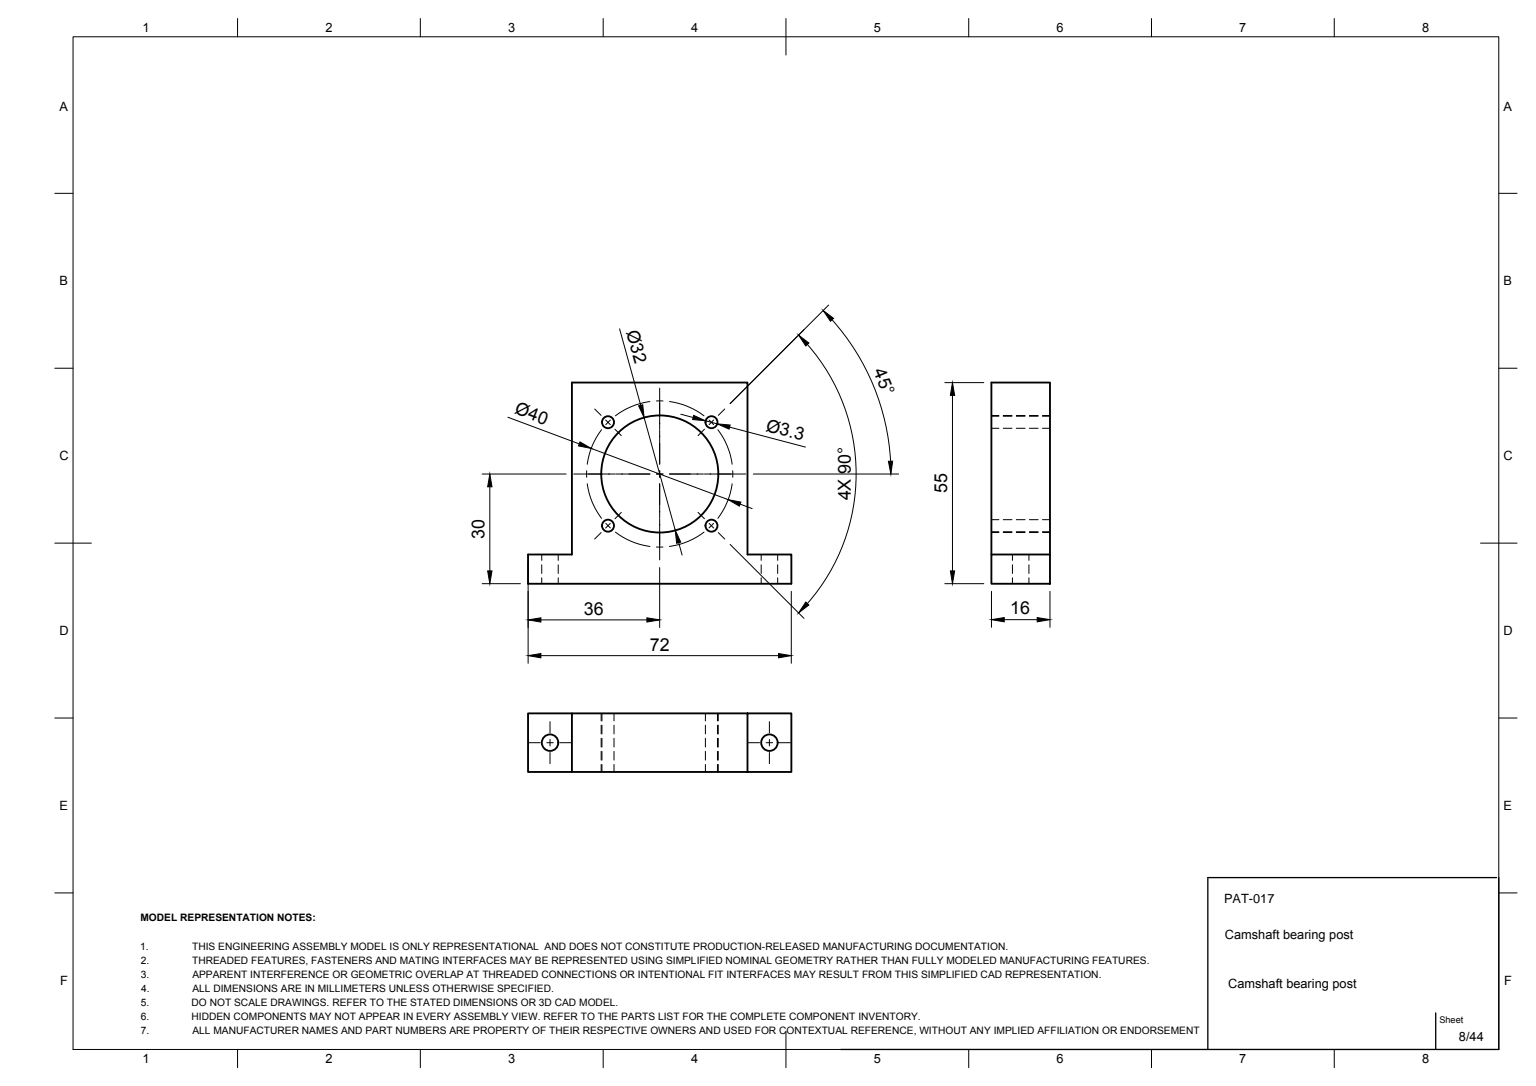
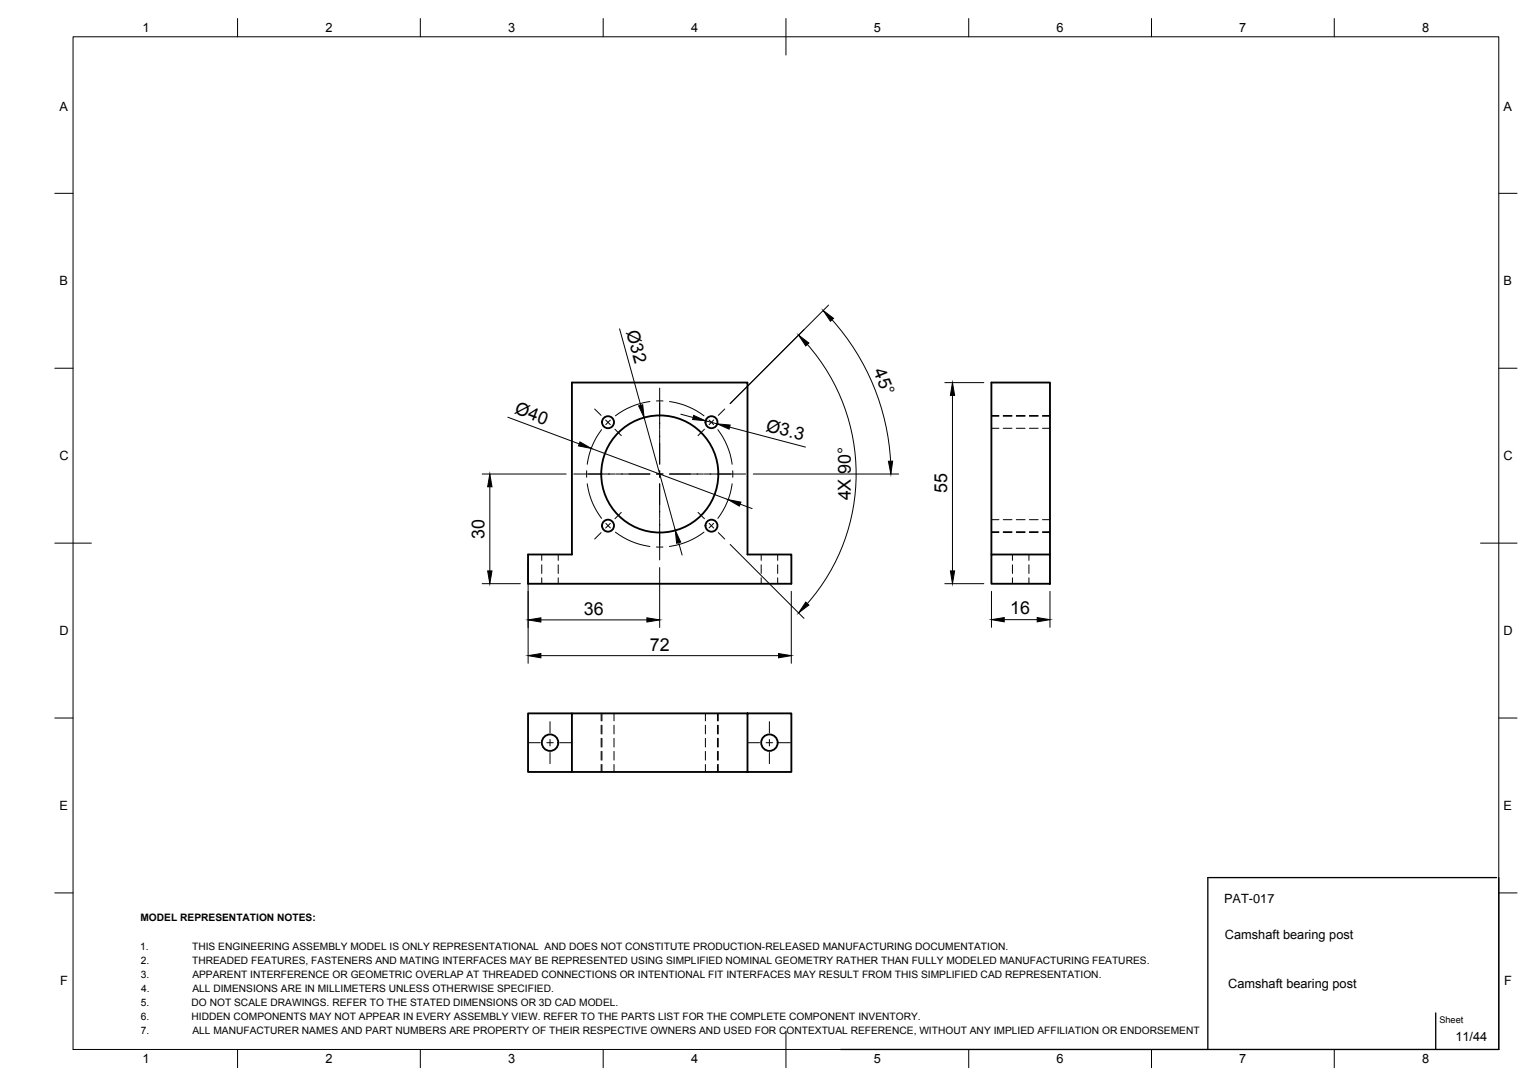
ISO-10303-21;
HEADER;
/* Generated by software containing ST-Developer
 * from STEP Tools, Inc. (www.steptools.com) 
 */

FILE_DESCRIPTION(
/* description */ ('Cam-and-follower valve demonstrator'),
/* implementation_level */ '2;1');

FILE_NAME(
/* name */ 'Camshaft bearing post.step',
/* time_stamp */ '2026-10-28T03:25:17-07:00',
/* author */ (''),
/* organization */ (''),
/* preprocessor_version */ 'ST-DEVELOPER v20.2',
/* originating_system */ 'Autodesk Translation Framework v15.17.0.0',
/* authorisation */ '');

FILE_SCHEMA (('AUTOMOTIVE_DESIGN { 1 0 10303 214 3 1 1 }'));
ENDSEC;

DATA;
#10=MECHANICAL_DESIGN_GEOMETRIC_PRESENTATION_REPRESENTATION('',(#415),#12896);
#343=SHAPE_REPRESENTATION_RELATIONSHIP('SRR','None',#13059,#379);
#379=ADVANCED_BREP_SHAPE_REPRESENTATION('',(#458),#12859);
#415=STYLED_ITEM('',(#13330),#458);
#458=MANIFOLD_SOLID_BREP('Body1',#6182);
#508=FACE_BOUND('',#1513,.T.);
#509=FACE_BOUND('',#1515,.T.);
#510=FACE_BOUND('',#1519,.T.);
#511=FACE_BOUND('',#1520,.T.);
#512=FACE_BOUND('',#1521,.T.);
#513=FACE_BOUND('',#1522,.T.);
#514=FACE_BOUND('',#1523,.T.);
#515=FACE_BOUND('',#1526,.T.);
#516=FACE_BOUND('',#1527,.T.);
#517=FACE_BOUND('',#1528,.T.);
#518=FACE_BOUND('',#1529,.T.);
#519=FACE_BOUND('',#1530,.T.);
#520=FACE_BOUND('',#1534,.T.);
#521=FACE_BOUND('',#1535,.T.);
#671=CIRCLE('',#6670,0.225);
#672=CIRCLE('',#6671,0.225);
#673=CIRCLE('',#6673,0.225);
#674=CIRCLE('',#6674,0.225);
#675=CIRCLE('',#6676,0.165);
#676=CIRCLE('',#6677,0.165);
#677=CIRCLE('',#6679,0.165);
#678=CIRCLE('',#6680,0.165);
#679=CIRCLE('',#6682,0.165);
#680=CIRCLE('',#6683,0.165);
#681=CIRCLE('',#6685,0.165);
#682=CIRCLE('',#6686,0.165);
#683=CIRCLE('',#6688,1.6);
#684=CIRCLE('',#6689,1.6);
#979=CYLINDRICAL_SURFACE('',#6669,0.225);
#980=CYLINDRICAL_SURFACE('',#6672,0.225);
#981=CYLINDRICAL_SURFACE('',#6675,0.165);
#982=CYLINDRICAL_SURFACE('',#6678,0.165);
#983=CYLINDRICAL_SURFACE('',#6681,0.165);
#984=CYLINDRICAL_SURFACE('',#6684,0.165);
#985=CYLINDRICAL_SURFACE('',#6687,1.6);
#1124=FACE_OUTER_BOUND('',#1505,.T.);
#1125=FACE_OUTER_BOUND('',#1506,.T.);
#1126=FACE_OUTER_BOUND('',#1507,.T.);
#1127=FACE_OUTER_BOUND('',#1508,.T.);
#1128=FACE_OUTER_BOUND('',#1509,.T.);
#1129=FACE_OUTER_BOUND('',#1510,.T.);
#1130=FACE_OUTER_BOUND('',#1511,.T.);
#1131=FACE_OUTER_BOUND('',#1512,.T.);
#1132=FACE_OUTER_BOUND('',#1514,.T.);
#1133=FACE_OUTER_BOUND('',#1516,.T.);
#1134=FACE_OUTER_BOUND('',#1517,.T.);
#1135=FACE_OUTER_BOUND('',#1518,.T.);
#1136=FACE_OUTER_BOUND('',#1524,.T.);
#1137=FACE_OUTER_BOUND('',#1525,.T.);
#1138=FACE_OUTER_BOUND('',#1531,.T.);
#1139=FACE_OUTER_BOUND('',#1532,.T.);
#1140=FACE_OUTER_BOUND('',#1533,.T.);
#1505=EDGE_LOOP('',(#4227,#4228,#4229,#4230));
#1506=EDGE_LOOP('',(#4231,#4232,#4233,#4234));
#1507=EDGE_LOOP('',(#4235,#4236,#4237,#4238));
#1508=EDGE_LOOP('',(#4239,#4240,#4241,#4242));
#1509=EDGE_LOOP('',(#4243,#4244,#4245,#4246));
#1510=EDGE_LOOP('',(#4247,#4248,#4249,#4250));
#1511=EDGE_LOOP('',(#4251,#4252,#4253,#4254));
#1512=EDGE_LOOP('',(#4255,#4256,#4257,#4258));
#1513=EDGE_LOOP('',(#4259));
#1514=EDGE_LOOP('',(#4260,#4261,#4262,#4263));
#1515=EDGE_LOOP('',(#4264));
#1516=EDGE_LOOP('',(#4265,#4266,#4267,#4268));
#1517=EDGE_LOOP('',(#4269,#4270,#4271,#4272));
#1518=EDGE_LOOP('',(#4273,#4274,#4275,#4276,#4277,#4278,#4279,#4280));
#1519=EDGE_LOOP('',(#4281));
#1520=EDGE_LOOP('',(#4282));
#1521=EDGE_LOOP('',(#4283));
#1522=EDGE_LOOP('',(#4284));
#1523=EDGE_LOOP('',(#4285));
#1524=EDGE_LOOP('',(#4286,#4287,#4288,#4289));
#1525=EDGE_LOOP('',(#4290,#4291,#4292,#4293,#4294,#4295,#4296,#4297));
#1526=EDGE_LOOP('',(#4298));
#1527=EDGE_LOOP('',(#4299));
#1528=EDGE_LOOP('',(#4300));
#1529=EDGE_LOOP('',(#4301));
#1530=EDGE_LOOP('',(#4302));
#1531=EDGE_LOOP('',(#4303,#4304,#4305,#4306));
#1532=EDGE_LOOP('',(#4307,#4308,#4309,#4310));
#1533=EDGE_LOOP('',(#4311,#4312,#4313,#4314));
#1534=EDGE_LOOP('',(#4315));
#1535=EDGE_LOOP('',(#4316));
#2049=LINE('',#9569,#2471);
#2050=LINE('',#9575,#2472);
#2051=LINE('',#9581,#2473);
#2052=LINE('',#9587,#2474);
#2053=LINE('',#9593,#2475);
#2054=LINE('',#9599,#2476);
#2055=LINE('',#9605,#2477);
#2056=LINE('',#9610,#2478);
#2057=LINE('',#9612,#2479);
#2058=LINE('',#9614,#2480);
#2059=LINE('',#9615,#2481);
#2060=LINE('',#9619,#2482);
#2061=LINE('',#9621,#2483);
#2062=LINE('',#9623,#2484);
#2063=LINE('',#9624,#2485);
#2064=LINE('',#9627,#2486);
#2065=LINE('',#9629,#2487);
#2066=LINE('',#9630,#2488);
#2067=LINE('',#9633,#2489);
#2068=LINE('',#9635,#2490);
#2069=LINE('',#9636,#2491);
#2070=LINE('',#9639,#2492);
#2071=LINE('',#9641,#2493);
#2072=LINE('',#9642,#2494);
#2073=LINE('',#9643,#2495);
#2074=LINE('',#9646,#2496);
#2075=LINE('',#9647,#2497);
#2076=LINE('',#9650,#2498);
#2077=LINE('',#9651,#2499);
#2078=LINE('',#9652,#2500);
#2079=LINE('',#9654,#2501);
#2471=VECTOR('',#7566,0.225);
#2472=VECTOR('',#7573,0.225);
#2473=VECTOR('',#7580,0.165);
#2474=VECTOR('',#7587,0.165);
#2475=VECTOR('',#7594,0.165);
#2476=VECTOR('',#7601,0.165);
#2477=VECTOR('',#7608,1.6);
#2478=VECTOR('',#7613,1.);
#2479=VECTOR('',#7614,1.);
#2480=VECTOR('',#7615,1.);
#2481=VECTOR('',#7616,1.);
#2482=VECTOR('',#7619,1.);
#2483=VECTOR('',#7620,1.);
#2484=VECTOR('',#7621,1.);
#2485=VECTOR('',#7622,1.);
#2486=VECTOR('',#7625,1.);
#2487=VECTOR('',#7626,1.);
#2488=VECTOR('',#7627,1.);
#2489=VECTOR('',#7630,1.);
#2490=VECTOR('',#7631,1.);
#2491=VECTOR('',#7632,1.);
#2492=VECTOR('',#7635,1.);
#2493=VECTOR('',#7636,1.);
#2494=VECTOR('',#7637,1.);
#2495=VECTOR('',#7638,1.);
#2496=VECTOR('',#7641,1.);
#2497=VECTOR('',#7642,1.);
#2498=VECTOR('',#7645,1.);
#2499=VECTOR('',#7646,1.);
#2500=VECTOR('',#7647,1.);
#2501=VECTOR('',#7650,1.);
#2883=VERTEX_POINT('',#9566);
#2884=VERTEX_POINT('',#9568);
#2885=VERTEX_POINT('',#9572);
#2886=VERTEX_POINT('',#9574);
#2887=VERTEX_POINT('',#9578);
#2888=VERTEX_POINT('',#9580);
#2889=VERTEX_POINT('',#9584);
#2890=VERTEX_POINT('',#9586);
#2891=VERTEX_POINT('',#9590);
#2892=VERTEX_POINT('',#9592);
#2893=VERTEX_POINT('',#9596);
#2894=VERTEX_POINT('',#9598);
#2895=VERTEX_POINT('',#9602);
#2896=VERTEX_POINT('',#9604);
#2897=VERTEX_POINT('',#9608);
#2898=VERTEX_POINT('',#9609);
#2899=VERTEX_POINT('',#9611);
#2900=VERTEX_POINT('',#9613);
#2901=VERTEX_POINT('',#9617);
#2902=VERTEX_POINT('',#9618);
#2903=VERTEX_POINT('',#9620);
#2904=VERTEX_POINT('',#9622);
#2905=VERTEX_POINT('',#9626);
#2906=VERTEX_POINT('',#9628);
#2907=VERTEX_POINT('',#9632);
#2908=VERTEX_POINT('',#9634);
#2909=VERTEX_POINT('',#9638);
#2910=VERTEX_POINT('',#9640);
#2911=VERTEX_POINT('',#9645);
#2912=VERTEX_POINT('',#9649);
#3410=EDGE_CURVE('',#2883,#2883,#671,.T.);
#3411=EDGE_CURVE('',#2883,#2884,#2049,.T.);
#3412=EDGE_CURVE('',#2884,#2884,#672,.T.);
#3413=EDGE_CURVE('',#2885,#2885,#673,.T.);
#3414=EDGE_CURVE('',#2885,#2886,#2050,.T.);
#3415=EDGE_CURVE('',#2886,#2886,#674,.T.);
#3416=EDGE_CURVE('',#2887,#2887,#675,.T.);
#3417=EDGE_CURVE('',#2887,#2888,#2051,.T.);
#3418=EDGE_CURVE('',#2888,#2888,#676,.T.);
#3419=EDGE_CURVE('',#2889,#2889,#677,.T.);
#3420=EDGE_CURVE('',#2889,#2890,#2052,.T.);
#3421=EDGE_CURVE('',#2890,#2890,#678,.T.);
#3422=EDGE_CURVE('',#2891,#2891,#679,.T.);
#3423=EDGE_CURVE('',#2891,#2892,#2053,.T.);
#3424=EDGE_CURVE('',#2892,#2892,#680,.T.);
#3425=EDGE_CURVE('',#2893,#2893,#681,.T.);
#3426=EDGE_CURVE('',#2893,#2894,#2054,.T.);
#3427=EDGE_CURVE('',#2894,#2894,#682,.T.);
#3428=EDGE_CURVE('',#2895,#2895,#683,.T.);
#3429=EDGE_CURVE('',#2895,#2896,#2055,.T.);
#3430=EDGE_CURVE('',#2896,#2896,#684,.T.);
#3431=EDGE_CURVE('',#2897,#2898,#2056,.T.);
#3432=EDGE_CURVE('',#2899,#2897,#2057,.T.);
#3433=EDGE_CURVE('',#2899,#2900,#2058,.T.);
#3434=EDGE_CURVE('',#2898,#2900,#2059,.T.);
#3435=EDGE_CURVE('',#2901,#2902,#2060,.T.);
#3436=EDGE_CURVE('',#2903,#2901,#2061,.T.);
#3437=EDGE_CURVE('',#2904,#2903,#2062,.T.);
#3438=EDGE_CURVE('',#2902,#2904,#2063,.T.);
#3439=EDGE_CURVE('',#2904,#2905,#2064,.T.);
#3440=EDGE_CURVE('',#2906,#2903,#2065,.T.);
#3441=EDGE_CURVE('',#2905,#2906,#2066,.T.);
#3442=EDGE_CURVE('',#2907,#2899,#2067,.T.);
#3443=EDGE_CURVE('',#2907,#2908,#2068,.T.);
#3444=EDGE_CURVE('',#2900,#2908,#2069,.T.);
#3445=EDGE_CURVE('',#2897,#2909,#2070,.T.);
#3446=EDGE_CURVE('',#2910,#2909,#2071,.T.);
#3447=EDGE_CURVE('',#2902,#2910,#2072,.T.);
#3448=EDGE_CURVE('',#2905,#2907,#2073,.T.);
#3449=EDGE_CURVE('',#2898,#2911,#2074,.T.);
#3450=EDGE_CURVE('',#2909,#2911,#2075,.T.);
#3451=EDGE_CURVE('',#2901,#2912,#2076,.T.);
#3452=EDGE_CURVE('',#2911,#2912,#2077,.T.);
#3453=EDGE_CURVE('',#2908,#2906,#2078,.T.);
#3454=EDGE_CURVE('',#2912,#2910,#2079,.T.);
#4227=ORIENTED_EDGE('',*,*,#3410,.F.);
#4228=ORIENTED_EDGE('',*,*,#3411,.T.);
#4229=ORIENTED_EDGE('',*,*,#3412,.F.);
#4230=ORIENTED_EDGE('',*,*,#3411,.F.);
#4231=ORIENTED_EDGE('',*,*,#3413,.F.);
#4232=ORIENTED_EDGE('',*,*,#3414,.T.);
#4233=ORIENTED_EDGE('',*,*,#3415,.F.);
#4234=ORIENTED_EDGE('',*,*,#3414,.F.);
#4235=ORIENTED_EDGE('',*,*,#3416,.F.);
#4236=ORIENTED_EDGE('',*,*,#3417,.T.);
#4237=ORIENTED_EDGE('',*,*,#3418,.F.);
#4238=ORIENTED_EDGE('',*,*,#3417,.F.);
#4239=ORIENTED_EDGE('',*,*,#3419,.F.);
#4240=ORIENTED_EDGE('',*,*,#3420,.T.);
#4241=ORIENTED_EDGE('',*,*,#3421,.F.);
#4242=ORIENTED_EDGE('',*,*,#3420,.F.);
#4243=ORIENTED_EDGE('',*,*,#3422,.F.);
#4244=ORIENTED_EDGE('',*,*,#3423,.T.);
#4245=ORIENTED_EDGE('',*,*,#3424,.F.);
#4246=ORIENTED_EDGE('',*,*,#3423,.F.);
#4247=ORIENTED_EDGE('',*,*,#3425,.F.);
#4248=ORIENTED_EDGE('',*,*,#3426,.T.);
#4249=ORIENTED_EDGE('',*,*,#3427,.F.);
#4250=ORIENTED_EDGE('',*,*,#3426,.F.);
#4251=ORIENTED_EDGE('',*,*,#3428,.F.);
#4252=ORIENTED_EDGE('',*,*,#3429,.T.);
#4253=ORIENTED_EDGE('',*,*,#3430,.F.);
#4254=ORIENTED_EDGE('',*,*,#3429,.F.);
#4255=ORIENTED_EDGE('',*,*,#3431,.F.);
#4256=ORIENTED_EDGE('',*,*,#3432,.F.);
#4257=ORIENTED_EDGE('',*,*,#3433,.T.);
#4258=ORIENTED_EDGE('',*,*,#3434,.F.);
#4259=ORIENTED_EDGE('',*,*,#3415,.T.);
#4260=ORIENTED_EDGE('',*,*,#3435,.F.);
#4261=ORIENTED_EDGE('',*,*,#3436,.F.);
#4262=ORIENTED_EDGE('',*,*,#3437,.F.);
#4263=ORIENTED_EDGE('',*,*,#3438,.F.);
#4264=ORIENTED_EDGE('',*,*,#3412,.T.);
#4265=ORIENTED_EDGE('',*,*,#3439,.F.);
#4266=ORIENTED_EDGE('',*,*,#3437,.T.);
#4267=ORIENTED_EDGE('',*,*,#3440,.F.);
#4268=ORIENTED_EDGE('',*,*,#3441,.F.);
#4269=ORIENTED_EDGE('',*,*,#3442,.F.);
#4270=ORIENTED_EDGE('',*,*,#3443,.T.);
#4271=ORIENTED_EDGE('',*,*,#3444,.F.);
#4272=ORIENTED_EDGE('',*,*,#3433,.F.);
#4273=ORIENTED_EDGE('',*,*,#3445,.T.);
#4274=ORIENTED_EDGE('',*,*,#3446,.F.);
#4275=ORIENTED_EDGE('',*,*,#3447,.F.);
#4276=ORIENTED_EDGE('',*,*,#3438,.T.);
#4277=ORIENTED_EDGE('',*,*,#3439,.T.);
#4278=ORIENTED_EDGE('',*,*,#3448,.T.);
#4279=ORIENTED_EDGE('',*,*,#3442,.T.);
#4280=ORIENTED_EDGE('',*,*,#3432,.T.);
#4281=ORIENTED_EDGE('',*,*,#3428,.T.);
#4282=ORIENTED_EDGE('',*,*,#3425,.T.);
#4283=ORIENTED_EDGE('',*,*,#3422,.T.);
#4284=ORIENTED_EDGE('',*,*,#3419,.T.);
#4285=ORIENTED_EDGE('',*,*,#3416,.T.);
#4286=ORIENTED_EDGE('',*,*,#3431,.T.);
#4287=ORIENTED_EDGE('',*,*,#3449,.T.);
#4288=ORIENTED_EDGE('',*,*,#3450,.F.);
#4289=ORIENTED_EDGE('',*,*,#3445,.F.);
#4290=ORIENTED_EDGE('',*,*,#3451,.T.);
#4291=ORIENTED_EDGE('',*,*,#3452,.F.);
#4292=ORIENTED_EDGE('',*,*,#3449,.F.);
#4293=ORIENTED_EDGE('',*,*,#3434,.T.);
#4294=ORIENTED_EDGE('',*,*,#3444,.T.);
#4295=ORIENTED_EDGE('',*,*,#3453,.T.);
#4296=ORIENTED_EDGE('',*,*,#3440,.T.);
#4297=ORIENTED_EDGE('',*,*,#3436,.T.);
#4298=ORIENTED_EDGE('',*,*,#3430,.T.);
#4299=ORIENTED_EDGE('',*,*,#3427,.T.);
#4300=ORIENTED_EDGE('',*,*,#3424,.T.);
#4301=ORIENTED_EDGE('',*,*,#3421,.T.);
#4302=ORIENTED_EDGE('',*,*,#3418,.T.);
#4303=ORIENTED_EDGE('',*,*,#3435,.T.);
#4304=ORIENTED_EDGE('',*,*,#3447,.T.);
#4305=ORIENTED_EDGE('',*,*,#3454,.F.);
#4306=ORIENTED_EDGE('',*,*,#3451,.F.);
#4307=ORIENTED_EDGE('',*,*,#3454,.T.);
#4308=ORIENTED_EDGE('',*,*,#3446,.T.);
#4309=ORIENTED_EDGE('',*,*,#3450,.T.);
#4310=ORIENTED_EDGE('',*,*,#3452,.T.);
#4311=ORIENTED_EDGE('',*,*,#3453,.F.);
#4312=ORIENTED_EDGE('',*,*,#3443,.F.);
#4313=ORIENTED_EDGE('',*,*,#3448,.F.);
#4314=ORIENTED_EDGE('',*,*,#3441,.T.);
#4315=ORIENTED_EDGE('',*,*,#3410,.T.);
#4316=ORIENTED_EDGE('',*,*,#3413,.T.);
#5620=PLANE('',#6690);
#5621=PLANE('',#6691);
#5622=PLANE('',#6692);
#5623=PLANE('',#6693);
#5624=PLANE('',#6694);
#5625=PLANE('',#6695);
#5626=PLANE('',#6696);
#5627=PLANE('',#6697);
#5628=PLANE('',#6698);
#5629=PLANE('',#6699);
#5840=ADVANCED_FACE('',(#1124),#979,.F.);
#5841=ADVANCED_FACE('',(#1125),#980,.F.);
#5842=ADVANCED_FACE('',(#1126),#981,.F.);
#5843=ADVANCED_FACE('',(#1127),#982,.F.);
#5844=ADVANCED_FACE('',(#1128),#983,.F.);
#5845=ADVANCED_FACE('',(#1129),#984,.F.);
#5846=ADVANCED_FACE('',(#1130),#985,.F.);
#5847=ADVANCED_FACE('',(#1131,#508),#5620,.T.);
#5848=ADVANCED_FACE('',(#1132,#509),#5621,.T.);
#5849=ADVANCED_FACE('',(#1133),#5622,.T.);
#5850=ADVANCED_FACE('',(#1134),#5623,.T.);
#5851=ADVANCED_FACE('',(#1135,#510,#511,#512,#513,#514),#5624,.T.);
#5852=ADVANCED_FACE('',(#1136),#5625,.T.);
#5853=ADVANCED_FACE('',(#1137,#515,#516,#517,#518,#519),#5626,.T.);
#5854=ADVANCED_FACE('',(#1138),#5627,.T.);
#5855=ADVANCED_FACE('',(#1139),#5628,.T.);
#5856=ADVANCED_FACE('',(#1140,#520,#521),#5629,.F.);
#6182=CLOSED_SHELL('',(#5840,#5841,#5842,#5843,#5844,#5845,#5846,#5847,
#5848,#5849,#5850,#5851,#5852,#5853,#5854,#5855,#5856));
#6668=AXIS2_PLACEMENT_3D('',#9564,#7560,#7561);
#6669=AXIS2_PLACEMENT_3D('',#9565,#7562,#7563);
#6670=AXIS2_PLACEMENT_3D('',#9567,#7564,#7565);
#6671=AXIS2_PLACEMENT_3D('',#9570,#7567,#7568);
#6672=AXIS2_PLACEMENT_3D('',#9571,#7569,#7570);
#6673=AXIS2_PLACEMENT_3D('',#9573,#7571,#7572);
#6674=AXIS2_PLACEMENT_3D('',#9576,#7574,#7575);
#6675=AXIS2_PLACEMENT_3D('',#9577,#7576,#7577);
#6676=AXIS2_PLACEMENT_3D('',#9579,#7578,#7579);
#6677=AXIS2_PLACEMENT_3D('',#9582,#7581,#7582);
#6678=AXIS2_PLACEMENT_3D('',#9583,#7583,#7584);
#6679=AXIS2_PLACEMENT_3D('',#9585,#7585,#7586);
#6680=AXIS2_PLACEMENT_3D('',#9588,#7588,#7589);
#6681=AXIS2_PLACEMENT_3D('',#9589,#7590,#7591);
#6682=AXIS2_PLACEMENT_3D('',#9591,#7592,#7593);
#6683=AXIS2_PLACEMENT_3D('',#9594,#7595,#7596);
#6684=AXIS2_PLACEMENT_3D('',#9595,#7597,#7598);
#6685=AXIS2_PLACEMENT_3D('',#9597,#7599,#7600);
#6686=AXIS2_PLACEMENT_3D('',#9600,#7602,#7603);
#6687=AXIS2_PLACEMENT_3D('',#9601,#7604,#7605);
#6688=AXIS2_PLACEMENT_3D('',#9603,#7606,#7607);
#6689=AXIS2_PLACEMENT_3D('',#9606,#7609,#7610);
#6690=AXIS2_PLACEMENT_3D('',#9607,#7611,#7612);
#6691=AXIS2_PLACEMENT_3D('',#9616,#7617,#7618);
#6692=AXIS2_PLACEMENT_3D('',#9625,#7623,#7624);
#6693=AXIS2_PLACEMENT_3D('',#9631,#7628,#7629);
#6694=AXIS2_PLACEMENT_3D('',#9637,#7633,#7634);
#6695=AXIS2_PLACEMENT_3D('',#9644,#7639,#7640);
#6696=AXIS2_PLACEMENT_3D('',#9648,#7643,#7644);
#6697=AXIS2_PLACEMENT_3D('',#9653,#7648,#7649);
#6698=AXIS2_PLACEMENT_3D('',#9655,#7651,#7652);
#6699=AXIS2_PLACEMENT_3D('',#9656,#7653,#7654);
#7560=DIRECTION('axis',(0.,0.,1.));
#7561=DIRECTION('refdir',(1.,0.,0.));
#7562=DIRECTION('center_axis',(0.,0.,1.));
#7563=DIRECTION('ref_axis',(1.,0.,0.));
#7564=DIRECTION('center_axis',(0.,0.,1.));
#7565=DIRECTION('ref_axis',(1.,0.,0.));
#7566=DIRECTION('',(0.,0.,1.));
#7567=DIRECTION('center_axis',(0.,0.,-1.));
#7568=DIRECTION('ref_axis',(1.,0.,0.));
#7569=DIRECTION('center_axis',(0.,0.,1.));
#7570=DIRECTION('ref_axis',(1.,0.,0.));
#7571=DIRECTION('center_axis',(0.,0.,1.));
#7572=DIRECTION('ref_axis',(1.,0.,0.));
#7573=DIRECTION('',(0.,0.,1.));
#7574=DIRECTION('center_axis',(0.,0.,-1.));
#7575=DIRECTION('ref_axis',(1.,0.,0.));
#7576=DIRECTION('center_axis',(0.,1.,0.));
#7577=DIRECTION('ref_axis',(1.,0.,0.));
#7578=DIRECTION('center_axis',(0.,1.,0.));
#7579=DIRECTION('ref_axis',(1.,0.,0.));
#7580=DIRECTION('',(0.,1.,0.));
#7581=DIRECTION('center_axis',(0.,-1.,0.));
#7582=DIRECTION('ref_axis',(1.,0.,0.));
#7583=DIRECTION('center_axis',(0.,1.,0.));
#7584=DIRECTION('ref_axis',(1.,0.,0.));
#7585=DIRECTION('center_axis',(0.,1.,0.));
#7586=DIRECTION('ref_axis',(1.,0.,0.));
#7587=DIRECTION('',(0.,1.,0.));
#7588=DIRECTION('center_axis',(0.,-1.,0.));
#7589=DIRECTION('ref_axis',(1.,0.,0.));
#7590=DIRECTION('center_axis',(0.,1.,0.));
#7591=DIRECTION('ref_axis',(1.,0.,0.));
#7592=DIRECTION('center_axis',(0.,1.,0.));
#7593=DIRECTION('ref_axis',(1.,0.,0.));
#7594=DIRECTION('',(0.,1.,0.));
#7595=DIRECTION('center_axis',(0.,-1.,0.));
#7596=DIRECTION('ref_axis',(1.,0.,0.));
#7597=DIRECTION('center_axis',(0.,1.,0.));
#7598=DIRECTION('ref_axis',(1.,0.,0.));
#7599=DIRECTION('center_axis',(0.,1.,0.));
#7600=DIRECTION('ref_axis',(1.,0.,0.));
#7601=DIRECTION('',(0.,1.,0.));
#7602=DIRECTION('center_axis',(0.,-1.,0.));
#7603=DIRECTION('ref_axis',(1.,0.,0.));
#7604=DIRECTION('center_axis',(0.,1.,0.));
#7605=DIRECTION('ref_axis',(1.,0.,0.));
#7606=DIRECTION('center_axis',(0.,1.,0.));
#7607=DIRECTION('ref_axis',(1.,0.,0.));
#7608=DIRECTION('',(0.,1.,0.));
#7609=DIRECTION('center_axis',(0.,-1.,0.));
#7610=DIRECTION('ref_axis',(1.,0.,0.));
#7611=DIRECTION('center_axis',(0.,0.,1.));
#7612=DIRECTION('ref_axis',(1.,0.,0.));
#7613=DIRECTION('',(0.,1.,0.));
#7614=DIRECTION('',(-1.,0.,0.));
#7615=DIRECTION('',(0.,1.,0.));
#7616=DIRECTION('',(1.,0.,0.));
#7617=DIRECTION('center_axis',(0.,0.,1.));
#7618=DIRECTION('ref_axis',(1.,0.,0.));
#7619=DIRECTION('',(0.,-1.,0.));
#7620=DIRECTION('',(1.,0.,0.));
#7621=DIRECTION('',(0.,1.,0.));
#7622=DIRECTION('',(-1.,0.,0.));
#7623=DIRECTION('center_axis',(-1.,0.,0.));
#7624=DIRECTION('ref_axis',(0.,0.,1.));
#7625=DIRECTION('',(0.,0.,-1.));
#7626=DIRECTION('',(0.,0.,1.));
#7627=DIRECTION('',(0.,1.,0.));
#7628=DIRECTION('center_axis',(1.,0.,0.));
#7629=DIRECTION('ref_axis',(0.,0.,-1.));
#7630=DIRECTION('',(0.,0.,1.));
#7631=DIRECTION('',(0.,1.,0.));
#7632=DIRECTION('',(0.,0.,-1.));
#7633=DIRECTION('center_axis',(0.,-1.,0.));
#7634=DIRECTION('ref_axis',(1.,0.,0.));
#7635=DIRECTION('',(0.,0.,1.));
#7636=DIRECTION('',(1.,0.,0.));
#7637=DIRECTION('',(0.,0.,1.));
#7638=DIRECTION('',(1.,0.,0.));
#7639=DIRECTION('center_axis',(1.,0.,0.));
#7640=DIRECTION('ref_axis',(0.,1.,0.));
#7641=DIRECTION('',(0.,0.,1.));
#7642=DIRECTION('',(0.,1.,0.));
#7643=DIRECTION('center_axis',(0.,1.,0.));
#7644=DIRECTION('ref_axis',(-1.,0.,0.));
#7645=DIRECTION('',(0.,0.,1.));
#7646=DIRECTION('',(-1.,0.,0.));
#7647=DIRECTION('',(-1.,0.,0.));
#7648=DIRECTION('center_axis',(-1.,0.,0.));
#7649=DIRECTION('ref_axis',(0.,-1.,0.));
#7650=DIRECTION('',(0.,-1.,0.));
#7651=DIRECTION('center_axis',(0.,0.,1.));
#7652=DIRECTION('ref_axis',(1.,0.,0.));
#7653=DIRECTION('center_axis',(0.,0.,1.));
#7654=DIRECTION('ref_axis',(1.,0.,0.));
#9564=CARTESIAN_POINT('',(0.,0.,0.));
#9565=CARTESIAN_POINT('Origin',(-3.,-2.5,0.9));
#9566=CARTESIAN_POINT('',(-3.225,-2.5,1.));
#9567=CARTESIAN_POINT('Origin',(-3.,-2.5,1.));
#9568=CARTESIAN_POINT('',(-3.225,-2.5,1.8));
#9569=CARTESIAN_POINT('',(-3.225,-2.5,0.9));
#9570=CARTESIAN_POINT('Origin',(-3.,-2.5,1.8));
#9571=CARTESIAN_POINT('Origin',(3.,-2.5,0.9));
#9572=CARTESIAN_POINT('',(2.775,-2.5,1.));
#9573=CARTESIAN_POINT('Origin',(3.,-2.5,1.));
#9574=CARTESIAN_POINT('',(2.775,-2.5,1.8));
#9575=CARTESIAN_POINT('',(2.775,-2.5,0.9));
#9576=CARTESIAN_POINT('Origin',(3.,-2.5,1.8));
#9577=CARTESIAN_POINT('Origin',(-1.4142135623731,-3.4,2.58578643762691));
#9578=CARTESIAN_POINT('',(-1.5792135623731,-3.3,2.58578643762691));
#9579=CARTESIAN_POINT('Origin',(-1.4142135623731,-3.3,2.58578643762691));
#9580=CARTESIAN_POINT('',(-1.5792135623731,-1.7,2.58578643762691));
#9581=CARTESIAN_POINT('',(-1.5792135623731,-3.4,2.58578643762691));
#9582=CARTESIAN_POINT('Origin',(-1.4142135623731,-1.7,2.58578643762691));
#9583=CARTESIAN_POINT('Origin',(-1.41421356237309,-3.4,5.41421356237309));
#9584=CARTESIAN_POINT('',(-1.57921356237309,-3.3,5.41421356237309));
#9585=CARTESIAN_POINT('Origin',(-1.41421356237309,-3.3,5.41421356237309));
#9586=CARTESIAN_POINT('',(-1.57921356237309,-1.7,5.41421356237309));
#9587=CARTESIAN_POINT('',(-1.57921356237309,-3.4,5.41421356237309));
#9588=CARTESIAN_POINT('Origin',(-1.41421356237309,-1.7,5.41421356237309));
#9589=CARTESIAN_POINT('Origin',(1.4142135623731,-3.4,5.41421356237309));
#9590=CARTESIAN_POINT('',(1.2492135623731,-3.3,5.41421356237309));
#9591=CARTESIAN_POINT('Origin',(1.4142135623731,-3.3,5.41421356237309));
#9592=CARTESIAN_POINT('',(1.2492135623731,-1.7,5.41421356237309));
#9593=CARTESIAN_POINT('',(1.2492135623731,-3.4,5.41421356237309));
#9594=CARTESIAN_POINT('Origin',(1.4142135623731,-1.7,5.41421356237309));
#9595=CARTESIAN_POINT('Origin',(1.41421356237309,-3.4,2.5857864376269));
#9596=CARTESIAN_POINT('',(1.24921356237309,-3.3,2.5857864376269));
#9597=CARTESIAN_POINT('Origin',(1.41421356237309,-3.3,2.5857864376269));
#9598=CARTESIAN_POINT('',(1.24921356237309,-1.7,2.5857864376269));
#9599=CARTESIAN_POINT('',(1.24921356237309,-3.4,2.5857864376269));
#9600=CARTESIAN_POINT('Origin',(1.41421356237309,-1.7,2.5857864376269));
#9601=CARTESIAN_POINT('Origin',(0.,-3.4,4.));
#9602=CARTESIAN_POINT('',(-1.6,-3.3,4.));
#9603=CARTESIAN_POINT('Origin',(0.,-3.3,4.));
#9604=CARTESIAN_POINT('',(-1.6,-1.7,4.));
#9605=CARTESIAN_POINT('',(-1.6,-3.4,4.));
#9606=CARTESIAN_POINT('Origin',(0.,-1.7,4.));
#9607=CARTESIAN_POINT('Origin',(-3.6,-3.3,1.8));
#9608=CARTESIAN_POINT('',(2.4,-3.3,1.8));
#9609=CARTESIAN_POINT('',(2.4,-1.7,1.8));
#9610=CARTESIAN_POINT('',(2.4,-3.3,1.8));
#9611=CARTESIAN_POINT('',(3.6,-3.3,1.8));
#9612=CARTESIAN_POINT('',(3.6,-3.3,1.8));
#9613=CARTESIAN_POINT('',(3.6,-1.7,1.8));
#9614=CARTESIAN_POINT('',(3.6,-3.3,1.8));
#9615=CARTESIAN_POINT('',(3.6,-1.7,1.8));
#9616=CARTESIAN_POINT('Origin',(-3.6,-3.3,1.8));
#9617=CARTESIAN_POINT('',(-2.4,-1.7,1.8));
#9618=CARTESIAN_POINT('',(-2.4,-3.3,1.8));
#9619=CARTESIAN_POINT('',(-2.4,-2.5,1.8));
#9620=CARTESIAN_POINT('',(-3.6,-1.7,1.8));
#9621=CARTESIAN_POINT('',(3.6,-1.7,1.8));
#9622=CARTESIAN_POINT('',(-3.6,-3.3,1.8));
#9623=CARTESIAN_POINT('',(-3.6,-3.3,1.8));
#9624=CARTESIAN_POINT('',(3.6,-3.3,1.8));
#9625=CARTESIAN_POINT('Origin',(-3.6,-3.3,1.));
#9626=CARTESIAN_POINT('',(-3.6,-3.3,1.));
#9627=CARTESIAN_POINT('',(-3.6,-3.3,1.8));
#9628=CARTESIAN_POINT('',(-3.6,-1.7,1.));
#9629=CARTESIAN_POINT('',(-3.6,-1.7,1.8));
#9630=CARTESIAN_POINT('',(-3.6,-3.3,1.));
#9631=CARTESIAN_POINT('Origin',(3.6,-3.3,1.8));
#9632=CARTESIAN_POINT('',(3.6,-3.3,1.));
#9633=CARTESIAN_POINT('',(3.6,-3.3,1.));
#9634=CARTESIAN_POINT('',(3.6,-1.7,1.));
#9635=CARTESIAN_POINT('',(3.6,-3.3,1.));
#9636=CARTESIAN_POINT('',(3.6,-1.7,1.));
#9637=CARTESIAN_POINT('Origin',(-2.4,-3.3,1.));
#9638=CARTESIAN_POINT('',(2.4,-3.3,6.5));
#9639=CARTESIAN_POINT('',(2.4,-3.3,1.));
#9640=CARTESIAN_POINT('',(-2.4,-3.3,6.5));
#9641=CARTESIAN_POINT('',(-2.4,-3.3,6.5));
#9642=CARTESIAN_POINT('',(-2.4,-3.3,1.));
#9643=CARTESIAN_POINT('',(-3.6,-3.3,1.));
#9644=CARTESIAN_POINT('Origin',(2.4,-3.3,1.));
#9645=CARTESIAN_POINT('',(2.4,-1.7,6.5));
#9646=CARTESIAN_POINT('',(2.4,-1.7,1.));
#9647=CARTESIAN_POINT('',(2.4,-3.3,6.5));
#9648=CARTESIAN_POINT('Origin',(2.4,-1.7,1.));
#9649=CARTESIAN_POINT('',(-2.4,-1.7,6.5));
#9650=CARTESIAN_POINT('',(-2.4,-1.7,1.));
#9651=CARTESIAN_POINT('',(2.4,-1.7,6.5));
#9652=CARTESIAN_POINT('',(-3.6,-1.7,1.));
#9653=CARTESIAN_POINT('Origin',(-2.4,-1.7,1.));
#9654=CARTESIAN_POINT('',(-2.4,-1.7,6.5));
#9655=CARTESIAN_POINT('Origin',(0.,-2.5,6.5));
#9656=CARTESIAN_POINT('Origin',(0.,-2.5,1.));
#12816=UNCERTAINTY_MEASURE_WITH_UNIT(LENGTH_MEASURE(0.001),#12897,
'DISTANCE_ACCURACY_VALUE',
'Maximum model space distance between geometric entities at asserted c
onnectivities');
#12853=UNCERTAINTY_MEASURE_WITH_UNIT(LENGTH_MEASURE(0.001),#12897,
'DISTANCE_ACCURACY_VALUE',
'Maximum model space distance between geometric entities at asserted c
onnectivities');
#12859=(
GEOMETRIC_REPRESENTATION_CONTEXT(3)
GLOBAL_UNCERTAINTY_ASSIGNED_CONTEXT((#12816))
GLOBAL_UNIT_ASSIGNED_CONTEXT((#12897,#12899,#12900))
REPRESENTATION_CONTEXT('','3D')
);
#12896=(
GEOMETRIC_REPRESENTATION_CONTEXT(3)
GLOBAL_UNCERTAINTY_ASSIGNED_CONTEXT((#12853))
GLOBAL_UNIT_ASSIGNED_CONTEXT((#12897,#12899,#12900))
REPRESENTATION_CONTEXT('','3D')
);
#12897=(
LENGTH_UNIT()
NAMED_UNIT(*)
SI_UNIT(.CENTI.,.METRE.)
);
#12899=(
NAMED_UNIT(*)
PLANE_ANGLE_UNIT()
SI_UNIT($,.RADIAN.)
);
#12900=(
NAMED_UNIT(*)
SI_UNIT($,.STERADIAN.)
SOLID_ANGLE_UNIT()
);
#12906=SHAPE_DEFINITION_REPRESENTATION(#12948,#13059);
#12948=PRODUCT_DEFINITION_SHAPE('',$,#13102);
#13059=SHAPE_REPRESENTATION('',(#6668),#12859);
#13096=PRODUCT_DEFINITION_CONTEXT('part definition',#13224,'design');
#13102=PRODUCT_DEFINITION('Camshaft bearing post',
'Camshaft bearing post',#13144,#13096);
#13144=PRODUCT_DEFINITION_FORMATION('',$,#13231);
#13224=APPLICATION_CONTEXT(
'Core Data for Automotive Mechanical Design Process');
#13225=PRODUCT_CONTEXT('part definition',#13224,'mechanical');
#13231=PRODUCT('Camshaft bearing post','Camshaft bearing post',
'Camshaft bearing post',(#13225));
#13324=COLOUR_RGB('Grey',0.48,0.52,0.57);
#13325=FILL_AREA_STYLE_COLOUR('',#13324);
#13326=FILL_AREA_STYLE('',(#13325));
#13327=SURFACE_STYLE_FILL_AREA(#13326);
#13328=SURFACE_SIDE_STYLE('',(#13327));
#13329=SURFACE_STYLE_USAGE(.BOTH.,#13328);
#13330=PRESENTATION_STYLE_ASSIGNMENT((#13329));
ENDSEC;
END-ISO-10303-21;
